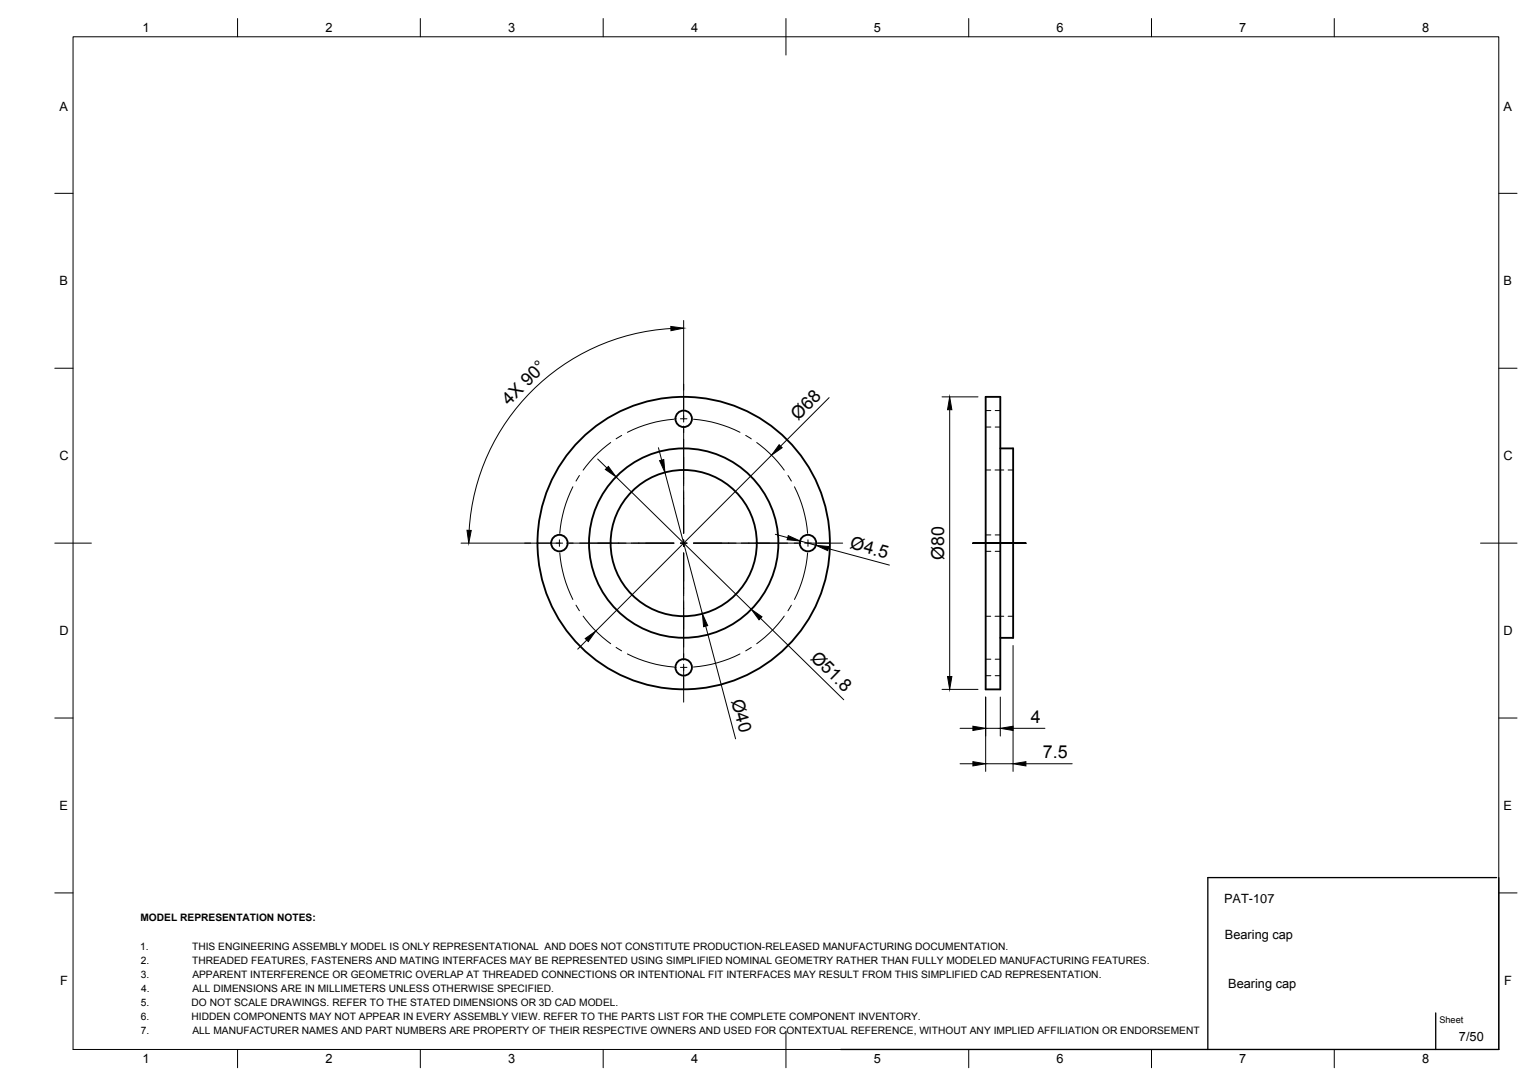
ISO-10303-21;
HEADER;
/* Generated by software containing ST-Developer
 * from STEP Tools, Inc. (www.steptools.com) 
 */

FILE_DESCRIPTION(
/* description */ ('Turntable on roller ring'),
/* implementation_level */ '2;1');

FILE_NAME(
/* name */ 'Bearing cap.step',
/* time_stamp */ '2026-10-28T03:23:59-07:00',
/* author */ (''),
/* organization */ (''),
/* preprocessor_version */ 'ST-DEVELOPER v20.2',
/* originating_system */ 'Autodesk Translation Framework v15.17.0.0',
/* authorisation */ '');

FILE_SCHEMA (('AUTOMOTIVE_DESIGN { 1 0 10303 214 3 1 1 }'));
ENDSEC;

DATA;
#10=MECHANICAL_DESIGN_GEOMETRIC_PRESENTATION_REPRESENTATION('',(#619),#16281);
#509=SHAPE_REPRESENTATION_RELATIONSHIP('SRR','None',#16523,#564);
#564=ADVANCED_BREP_SHAPE_REPRESENTATION('',(#691),#16217);
#619=STYLED_ITEM('',(#16932),#691);
#691=MANIFOLD_SOLID_BREP('Body1',#8360);
#812=FACE_BOUND('',#1872,.T.);
#813=FACE_BOUND('',#1876,.T.);
#814=FACE_BOUND('',#1877,.T.);
#815=FACE_BOUND('',#1878,.T.);
#816=FACE_BOUND('',#1879,.T.);
#817=FACE_BOUND('',#1880,.T.);
#818=FACE_BOUND('',#1882,.T.);
#819=FACE_BOUND('',#1883,.T.);
#820=FACE_BOUND('',#1884,.T.);
#821=FACE_BOUND('',#1885,.T.);
#822=FACE_BOUND('',#1886,.T.);
#1007=PLANE('',#9197);
#1008=PLANE('',#9204);
#1009=PLANE('',#9205);
#1306=FACE_OUTER_BOUND('',#1866,.T.);
#1307=FACE_OUTER_BOUND('',#1867,.T.);
#1308=FACE_OUTER_BOUND('',#1868,.T.);
#1309=FACE_OUTER_BOUND('',#1869,.T.);
#1310=FACE_OUTER_BOUND('',#1870,.T.);
#1311=FACE_OUTER_BOUND('',#1871,.T.);
#1312=FACE_OUTER_BOUND('',#1873,.T.);
#1313=FACE_OUTER_BOUND('',#1874,.T.);
#1314=FACE_OUTER_BOUND('',#1875,.T.);
#1315=FACE_OUTER_BOUND('',#1881,.T.);
#1866=EDGE_LOOP('',(#5917,#5918,#5919,#5920));
#1867=EDGE_LOOP('',(#5921,#5922,#5923,#5924));
#1868=EDGE_LOOP('',(#5925,#5926,#5927,#5928));
#1869=EDGE_LOOP('',(#5929,#5930,#5931,#5932));
#1870=EDGE_LOOP('',(#5933,#5934,#5935,#5936));
#1871=EDGE_LOOP('',(#5937));
#1872=EDGE_LOOP('',(#5938));
#1873=EDGE_LOOP('',(#5939,#5940,#5941,#5942));
#1874=EDGE_LOOP('',(#5943,#5944,#5945,#5946));
#1875=EDGE_LOOP('',(#5947));
#1876=EDGE_LOOP('',(#5948));
#1877=EDGE_LOOP('',(#5949));
#1878=EDGE_LOOP('',(#5950));
#1879=EDGE_LOOP('',(#5951));
#1880=EDGE_LOOP('',(#5952));
#1881=EDGE_LOOP('',(#5953));
#1882=EDGE_LOOP('',(#5954));
#1883=EDGE_LOOP('',(#5955));
#1884=EDGE_LOOP('',(#5956));
#1885=EDGE_LOOP('',(#5957));
#1886=EDGE_LOOP('',(#5958));
#2548=LINE('',#13289,#3031);
#2549=LINE('',#13295,#3032);
#2550=LINE('',#13301,#3033);
#2551=LINE('',#13307,#3034);
#2552=LINE('',#13313,#3035);
#2553=LINE('',#13321,#3036);
#2554=LINE('',#13326,#3037);
#3031=VECTOR('',#10543,0.225);
#3032=VECTOR('',#10550,0.225);
#3033=VECTOR('',#10557,0.225);
#3034=VECTOR('',#10564,0.225);
#3035=VECTOR('',#10571,2.59);
#3036=VECTOR('',#10582,2.);
#3037=VECTOR('',#10587,4.);
#3540=CIRCLE('',#9183,0.225);
#3541=CIRCLE('',#9184,0.225);
#3542=CIRCLE('',#9186,0.225);
#3543=CIRCLE('',#9187,0.225);
#3544=CIRCLE('',#9189,0.225);
#3545=CIRCLE('',#9190,0.225);
#3546=CIRCLE('',#9192,0.225);
#3547=CIRCLE('',#9193,0.225);
#3548=CIRCLE('',#9195,2.59);
#3549=CIRCLE('',#9196,2.59);
#3550=CIRCLE('',#9198,2.);
#3551=CIRCLE('',#9200,2.);
#3552=CIRCLE('',#9202,4.);
#3553=CIRCLE('',#9203,4.);
#4034=VERTEX_POINT('',#13286);
#4035=VERTEX_POINT('',#13288);
#4036=VERTEX_POINT('',#13292);
#4037=VERTEX_POINT('',#13294);
#4038=VERTEX_POINT('',#13298);
#4039=VERTEX_POINT('',#13300);
#4040=VERTEX_POINT('',#13304);
#4041=VERTEX_POINT('',#13306);
#4042=VERTEX_POINT('',#13310);
#4043=VERTEX_POINT('',#13312);
#4044=VERTEX_POINT('',#13316);
#4045=VERTEX_POINT('',#13319);
#4046=VERTEX_POINT('',#13323);
#4047=VERTEX_POINT('',#13325);
#4769=EDGE_CURVE('',#4034,#4034,#3540,.T.);
#4770=EDGE_CURVE('',#4034,#4035,#2548,.T.);
#4771=EDGE_CURVE('',#4035,#4035,#3541,.T.);
#4772=EDGE_CURVE('',#4036,#4036,#3542,.T.);
#4773=EDGE_CURVE('',#4036,#4037,#2549,.T.);
#4774=EDGE_CURVE('',#4037,#4037,#3543,.T.);
#4775=EDGE_CURVE('',#4038,#4038,#3544,.T.);
#4776=EDGE_CURVE('',#4038,#4039,#2550,.T.);
#4777=EDGE_CURVE('',#4039,#4039,#3545,.T.);
#4778=EDGE_CURVE('',#4040,#4040,#3546,.T.);
#4779=EDGE_CURVE('',#4040,#4041,#2551,.T.);
#4780=EDGE_CURVE('',#4041,#4041,#3547,.T.);
#4781=EDGE_CURVE('',#4042,#4042,#3548,.T.);
#4782=EDGE_CURVE('',#4042,#4043,#2552,.T.);
#4783=EDGE_CURVE('',#4043,#4043,#3549,.T.);
#4784=EDGE_CURVE('',#4044,#4044,#3550,.T.);
#4785=EDGE_CURVE('',#4045,#4045,#3551,.T.);
#4786=EDGE_CURVE('',#4045,#4044,#2553,.T.);
#4787=EDGE_CURVE('',#4046,#4046,#3552,.T.);
#4788=EDGE_CURVE('',#4046,#4047,#2554,.T.);
#4789=EDGE_CURVE('',#4047,#4047,#3553,.T.);
#5917=ORIENTED_EDGE('',*,*,#4769,.F.);
#5918=ORIENTED_EDGE('',*,*,#4770,.T.);
#5919=ORIENTED_EDGE('',*,*,#4771,.F.);
#5920=ORIENTED_EDGE('',*,*,#4770,.F.);
#5921=ORIENTED_EDGE('',*,*,#4772,.F.);
#5922=ORIENTED_EDGE('',*,*,#4773,.T.);
#5923=ORIENTED_EDGE('',*,*,#4774,.F.);
#5924=ORIENTED_EDGE('',*,*,#4773,.F.);
#5925=ORIENTED_EDGE('',*,*,#4775,.F.);
#5926=ORIENTED_EDGE('',*,*,#4776,.T.);
#5927=ORIENTED_EDGE('',*,*,#4777,.F.);
#5928=ORIENTED_EDGE('',*,*,#4776,.F.);
#5929=ORIENTED_EDGE('',*,*,#4778,.F.);
#5930=ORIENTED_EDGE('',*,*,#4779,.T.);
#5931=ORIENTED_EDGE('',*,*,#4780,.F.);
#5932=ORIENTED_EDGE('',*,*,#4779,.F.);
#5933=ORIENTED_EDGE('',*,*,#4781,.F.);
#5934=ORIENTED_EDGE('',*,*,#4782,.T.);
#5935=ORIENTED_EDGE('',*,*,#4783,.T.);
#5936=ORIENTED_EDGE('',*,*,#4782,.F.);
#5937=ORIENTED_EDGE('',*,*,#4783,.F.);
#5938=ORIENTED_EDGE('',*,*,#4784,.F.);
#5939=ORIENTED_EDGE('',*,*,#4785,.F.);
#5940=ORIENTED_EDGE('',*,*,#4786,.T.);
#5941=ORIENTED_EDGE('',*,*,#4784,.T.);
#5942=ORIENTED_EDGE('',*,*,#4786,.F.);
#5943=ORIENTED_EDGE('',*,*,#4787,.F.);
#5944=ORIENTED_EDGE('',*,*,#4788,.T.);
#5945=ORIENTED_EDGE('',*,*,#4789,.T.);
#5946=ORIENTED_EDGE('',*,*,#4788,.F.);
#5947=ORIENTED_EDGE('',*,*,#4787,.T.);
#5948=ORIENTED_EDGE('',*,*,#4785,.T.);
#5949=ORIENTED_EDGE('',*,*,#4780,.T.);
#5950=ORIENTED_EDGE('',*,*,#4777,.T.);
#5951=ORIENTED_EDGE('',*,*,#4774,.T.);
#5952=ORIENTED_EDGE('',*,*,#4771,.T.);
#5953=ORIENTED_EDGE('',*,*,#4789,.F.);
#5954=ORIENTED_EDGE('',*,*,#4781,.T.);
#5955=ORIENTED_EDGE('',*,*,#4778,.T.);
#5956=ORIENTED_EDGE('',*,*,#4775,.T.);
#5957=ORIENTED_EDGE('',*,*,#4772,.T.);
#5958=ORIENTED_EDGE('',*,*,#4769,.T.);
#7708=CYLINDRICAL_SURFACE('',#9182,0.225);
#7709=CYLINDRICAL_SURFACE('',#9185,0.225);
#7710=CYLINDRICAL_SURFACE('',#9188,0.225);
#7711=CYLINDRICAL_SURFACE('',#9191,0.225);
#7712=CYLINDRICAL_SURFACE('',#9194,2.59);
#7713=CYLINDRICAL_SURFACE('',#9199,2.);
#7714=CYLINDRICAL_SURFACE('',#9201,4.);
#7909=ADVANCED_FACE('',(#1306),#7708,.F.);
#7910=ADVANCED_FACE('',(#1307),#7709,.F.);
#7911=ADVANCED_FACE('',(#1308),#7710,.F.);
#7912=ADVANCED_FACE('',(#1309),#7711,.F.);
#7913=ADVANCED_FACE('',(#1310),#7712,.T.);
#7914=ADVANCED_FACE('',(#1311,#812),#1007,.F.);
#7915=ADVANCED_FACE('',(#1312),#7713,.F.);
#7916=ADVANCED_FACE('',(#1313),#7714,.T.);
#7917=ADVANCED_FACE('',(#1314,#813,#814,#815,#816,#817),#1008,.T.);
#7918=ADVANCED_FACE('',(#1315,#818,#819,#820,#821,#822),#1009,.F.);
#8360=CLOSED_SHELL('',(#7909,#7910,#7911,#7912,#7913,#7914,#7915,#7916,
#7917,#7918));
#9181=AXIS2_PLACEMENT_3D('',#13284,#10537,#10538);
#9182=AXIS2_PLACEMENT_3D('',#13285,#10539,#10540);
#9183=AXIS2_PLACEMENT_3D('',#13287,#10541,#10542);
#9184=AXIS2_PLACEMENT_3D('',#13290,#10544,#10545);
#9185=AXIS2_PLACEMENT_3D('',#13291,#10546,#10547);
#9186=AXIS2_PLACEMENT_3D('',#13293,#10548,#10549);
#9187=AXIS2_PLACEMENT_3D('',#13296,#10551,#10552);
#9188=AXIS2_PLACEMENT_3D('',#13297,#10553,#10554);
#9189=AXIS2_PLACEMENT_3D('',#13299,#10555,#10556);
#9190=AXIS2_PLACEMENT_3D('',#13302,#10558,#10559);
#9191=AXIS2_PLACEMENT_3D('',#13303,#10560,#10561);
#9192=AXIS2_PLACEMENT_3D('',#13305,#10562,#10563);
#9193=AXIS2_PLACEMENT_3D('',#13308,#10565,#10566);
#9194=AXIS2_PLACEMENT_3D('',#13309,#10567,#10568);
#9195=AXIS2_PLACEMENT_3D('',#13311,#10569,#10570);
#9196=AXIS2_PLACEMENT_3D('',#13314,#10572,#10573);
#9197=AXIS2_PLACEMENT_3D('',#13315,#10574,#10575);
#9198=AXIS2_PLACEMENT_3D('',#13317,#10576,#10577);
#9199=AXIS2_PLACEMENT_3D('',#13318,#10578,#10579);
#9200=AXIS2_PLACEMENT_3D('',#13320,#10580,#10581);
#9201=AXIS2_PLACEMENT_3D('',#13322,#10583,#10584);
#9202=AXIS2_PLACEMENT_3D('',#13324,#10585,#10586);
#9203=AXIS2_PLACEMENT_3D('',#13327,#10588,#10589);
#9204=AXIS2_PLACEMENT_3D('',#13328,#10590,#10591);
#9205=AXIS2_PLACEMENT_3D('',#13329,#10592,#10593);
#10537=DIRECTION('axis',(0.,0.,1.));
#10538=DIRECTION('refdir',(1.,0.,0.));
#10539=DIRECTION('center_axis',(0.,0.,1.));
#10540=DIRECTION('ref_axis',(1.,0.,0.));
#10541=DIRECTION('center_axis',(0.,0.,1.));
#10542=DIRECTION('ref_axis',(1.,0.,0.));
#10543=DIRECTION('',(0.,0.,1.));
#10544=DIRECTION('center_axis',(0.,0.,-1.));
#10545=DIRECTION('ref_axis',(1.,0.,0.));
#10546=DIRECTION('center_axis',(0.,0.,1.));
#10547=DIRECTION('ref_axis',(1.,0.,0.));
#10548=DIRECTION('center_axis',(0.,0.,1.));
#10549=DIRECTION('ref_axis',(1.,0.,0.));
#10550=DIRECTION('',(0.,0.,1.));
#10551=DIRECTION('center_axis',(0.,0.,-1.));
#10552=DIRECTION('ref_axis',(1.,0.,0.));
#10553=DIRECTION('center_axis',(0.,0.,1.));
#10554=DIRECTION('ref_axis',(1.,0.,0.));
#10555=DIRECTION('center_axis',(0.,0.,1.));
#10556=DIRECTION('ref_axis',(1.,0.,0.));
#10557=DIRECTION('',(0.,0.,1.));
#10558=DIRECTION('center_axis',(0.,0.,-1.));
#10559=DIRECTION('ref_axis',(1.,0.,0.));
#10560=DIRECTION('center_axis',(0.,0.,1.));
#10561=DIRECTION('ref_axis',(1.,0.,0.));
#10562=DIRECTION('center_axis',(0.,0.,1.));
#10563=DIRECTION('ref_axis',(1.,0.,0.));
#10564=DIRECTION('',(0.,0.,1.));
#10565=DIRECTION('center_axis',(0.,0.,-1.));
#10566=DIRECTION('ref_axis',(1.,0.,0.));
#10567=DIRECTION('center_axis',(0.,0.,1.));
#10568=DIRECTION('ref_axis',(1.,0.,0.));
#10569=DIRECTION('center_axis',(0.,0.,1.));
#10570=DIRECTION('ref_axis',(1.,0.,0.));
#10571=DIRECTION('',(0.,0.,-1.));
#10572=DIRECTION('center_axis',(0.,0.,1.));
#10573=DIRECTION('ref_axis',(1.,0.,0.));
#10574=DIRECTION('center_axis',(0.,0.,1.));
#10575=DIRECTION('ref_axis',(1.,0.,0.));
#10576=DIRECTION('center_axis',(0.,0.,-1.));
#10577=DIRECTION('ref_axis',(1.,0.,0.));
#10578=DIRECTION('center_axis',(0.,0.,1.));
#10579=DIRECTION('ref_axis',(1.,0.,0.));
#10580=DIRECTION('center_axis',(0.,0.,-1.));
#10581=DIRECTION('ref_axis',(1.,0.,0.));
#10582=DIRECTION('',(0.,0.,-1.));
#10583=DIRECTION('center_axis',(0.,0.,1.));
#10584=DIRECTION('ref_axis',(1.,0.,0.));
#10585=DIRECTION('center_axis',(0.,0.,1.));
#10586=DIRECTION('ref_axis',(1.,0.,0.));
#10587=DIRECTION('',(0.,0.,-1.));
#10588=DIRECTION('center_axis',(0.,0.,1.));
#10589=DIRECTION('ref_axis',(1.,0.,0.));
#10590=DIRECTION('center_axis',(0.,0.,1.));
#10591=DIRECTION('ref_axis',(1.,0.,0.));
#10592=DIRECTION('center_axis',(0.,0.,1.));
#10593=DIRECTION('ref_axis',(1.,0.,0.));
#13284=CARTESIAN_POINT('',(0.,0.,0.));
#13285=CARTESIAN_POINT('Origin',(-3.4,4.163799117101E-16,4.5));
#13286=CARTESIAN_POINT('',(-3.625,3.88825358729285E-16,4.6));
#13287=CARTESIAN_POINT('Origin',(-3.4,4.163799117101E-16,4.6));
#13288=CARTESIAN_POINT('',(-3.625,4.43934464690916E-16,5.));
#13289=CARTESIAN_POINT('',(-3.625,3.88825358729285E-16,4.5));
#13290=CARTESIAN_POINT('Origin',(-3.4,4.163799117101E-16,5.));
#13291=CARTESIAN_POINT('Origin',(2.0818995585505E-16,3.4,4.5));
#13292=CARTESIAN_POINT('',(-0.225,3.4,4.6));
#13293=CARTESIAN_POINT('Origin',(2.0818995585505E-16,3.4,4.6));
#13294=CARTESIAN_POINT('',(-0.225,3.4,5.));
#13295=CARTESIAN_POINT('',(-0.225,3.4,4.5));
#13296=CARTESIAN_POINT('Origin',(2.0818995585505E-16,3.4,5.));
#13297=CARTESIAN_POINT('Origin',(3.4,0.,4.5));
#13298=CARTESIAN_POINT('',(3.175,-2.75545529808155E-17,4.6));
#13299=CARTESIAN_POINT('Origin',(3.4,0.,4.6));
#13300=CARTESIAN_POINT('',(3.175,2.75545529808155E-17,5.));
#13301=CARTESIAN_POINT('',(3.175,-2.75545529808155E-17,4.5));
#13302=CARTESIAN_POINT('Origin',(3.4,0.,5.));
#13303=CARTESIAN_POINT('Origin',(-6.2456986756515E-16,-3.4,4.5));
#13304=CARTESIAN_POINT('',(-0.225000000000001,-3.4,4.6));
#13305=CARTESIAN_POINT('Origin',(-6.2456986756515E-16,-3.4,4.6));
#13306=CARTESIAN_POINT('',(-0.225000000000001,-3.4,5.));
#13307=CARTESIAN_POINT('',(-0.225000000000001,-3.4,4.5));
#13308=CARTESIAN_POINT('Origin',(-6.2456986756515E-16,-3.4,5.));
#13309=CARTESIAN_POINT('Origin',(0.,0.,4.25));
#13310=CARTESIAN_POINT('',(-2.59,-3.17183520979164E-16,4.6));
#13311=CARTESIAN_POINT('Origin',(0.,0.,4.6));
#13312=CARTESIAN_POINT('',(-2.59,-3.17183520979164E-16,4.25));
#13313=CARTESIAN_POINT('',(-2.59,-3.17183520979164E-16,4.25));
#13314=CARTESIAN_POINT('Origin',(0.,0.,4.25));
#13315=CARTESIAN_POINT('Origin',(0.,0.,4.25));
#13316=CARTESIAN_POINT('',(-2.,-2.44929359829471E-16,4.25));
#13317=CARTESIAN_POINT('Origin',(0.,0.,4.25));
#13318=CARTESIAN_POINT('Origin',(0.,0.,4.6));
#13319=CARTESIAN_POINT('',(-2.,-2.44929359829471E-16,5.));
#13320=CARTESIAN_POINT('Origin',(0.,0.,5.));
#13321=CARTESIAN_POINT('',(-2.,-2.44929359829471E-16,4.6));
#13322=CARTESIAN_POINT('Origin',(0.,0.,4.6));
#13323=CARTESIAN_POINT('',(-4.,-4.89858719658941E-16,5.));
#13324=CARTESIAN_POINT('Origin',(0.,0.,5.));
#13325=CARTESIAN_POINT('',(-4.,-4.89858719658941E-16,4.6));
#13326=CARTESIAN_POINT('',(-4.,-4.89858719658941E-16,4.6));
#13327=CARTESIAN_POINT('Origin',(0.,0.,4.6));
#13328=CARTESIAN_POINT('Origin',(0.,0.,5.));
#13329=CARTESIAN_POINT('Origin',(0.,0.,4.6));
#16148=UNCERTAINTY_MEASURE_WITH_UNIT(LENGTH_MEASURE(0.001),#16282,
'DISTANCE_ACCURACY_VALUE',
'Maximum model space distance between geometric entities at asserted c
onnectivities');
#16212=UNCERTAINTY_MEASURE_WITH_UNIT(LENGTH_MEASURE(0.001),#16282,
'DISTANCE_ACCURACY_VALUE',
'Maximum model space distance between geometric entities at asserted c
onnectivities');
#16217=(
GEOMETRIC_REPRESENTATION_CONTEXT(3)
GLOBAL_UNCERTAINTY_ASSIGNED_CONTEXT((#16148))
GLOBAL_UNIT_ASSIGNED_CONTEXT((#16282,#16284,#16285))
REPRESENTATION_CONTEXT('','3D')
);
#16281=(
GEOMETRIC_REPRESENTATION_CONTEXT(3)
GLOBAL_UNCERTAINTY_ASSIGNED_CONTEXT((#16212))
GLOBAL_UNIT_ASSIGNED_CONTEXT((#16282,#16284,#16285))
REPRESENTATION_CONTEXT('','3D')
);
#16282=(
LENGTH_UNIT()
NAMED_UNIT(*)
SI_UNIT(.CENTI.,.METRE.)
);
#16284=(
NAMED_UNIT(*)
PLANE_ANGLE_UNIT()
SI_UNIT($,.RADIAN.)
);
#16285=(
NAMED_UNIT(*)
SI_UNIT($,.STERADIAN.)
SOLID_ANGLE_UNIT()
);
#16290=SHAPE_DEFINITION_REPRESENTATION(#16358,#16523);
#16358=PRODUCT_DEFINITION_SHAPE('',$,#16592);
#16523=SHAPE_REPRESENTATION('',(#9181),#16217);
#16587=PRODUCT_DEFINITION_CONTEXT('part definition',#16793,'design');
#16592=PRODUCT_DEFINITION('Bearing cap','Bearing cap',#16660,#16587);
#16660=PRODUCT_DEFINITION_FORMATION('',$,#16799);
#16793=APPLICATION_CONTEXT(
'Core Data for Automotive Mechanical Design Process');
#16794=PRODUCT_CONTEXT('part definition',#16793,'mechanical');
#16799=PRODUCT('Bearing cap','Bearing cap','Bearing cap',(#16794));
#16926=COLOUR_RGB('Grey',0.48,0.52,0.57);
#16927=FILL_AREA_STYLE_COLOUR('',#16926);
#16928=FILL_AREA_STYLE('',(#16927));
#16929=SURFACE_STYLE_FILL_AREA(#16928);
#16930=SURFACE_SIDE_STYLE('',(#16929));
#16931=SURFACE_STYLE_USAGE(.BOTH.,#16930);
#16932=PRESENTATION_STYLE_ASSIGNMENT((#16931));
ENDSEC;
END-ISO-10303-21;
